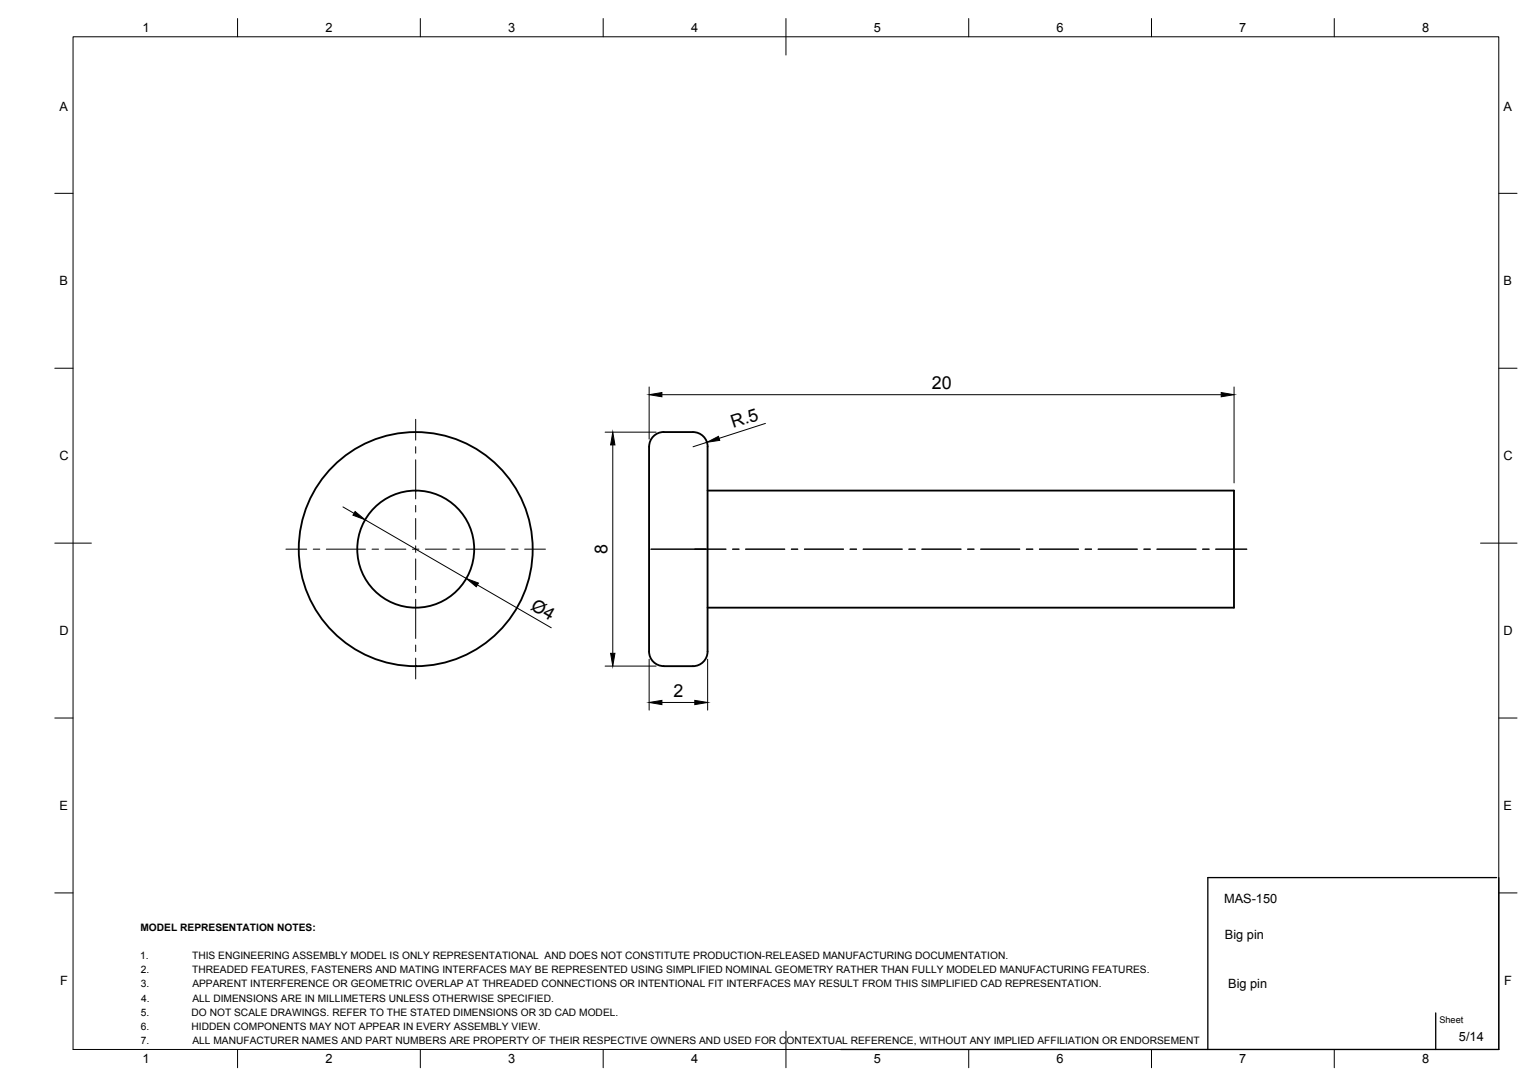
ISO-10303-21;
HEADER;
/* Generated by software containing ST-Developer
 * from STEP Tools, Inc. (www.steptools.com) 
 */

FILE_DESCRIPTION(
/* description */ ('STEP AP203'),
/* implementation_level */ '2;1');

FILE_NAME(
/* name */ 'Big pin.step',
/* time_stamp */ '2026-11-08T21:40:52-08:00',
/* author */ (''),
/* organization */ (''),
/* preprocessor_version */ 'ST-DEVELOPER v20.2',
/* originating_system */ 'Autodesk Translation Framework v15.17.0.0',
/* authorisation */ '');

FILE_SCHEMA (('AUTOMOTIVE_DESIGN { 1 0 10303 214 3 1 1 }'));
ENDSEC;

DATA;
#10=MECHANICAL_DESIGN_GEOMETRIC_PRESENTATION_REPRESENTATION('',(#192),#12137);
#170=SHAPE_REPRESENTATION_RELATIONSHIP('SRR','None',#12194,#181);
#181=ADVANCED_BREP_SHAPE_REPRESENTATION('',(#203),#12135);
#192=STYLED_ITEM('',(#12253),#203);
#203=MANIFOLD_SOLID_BREP('Body1',#1837);
#227=FACE_BOUND('',#723,.T.);
#269=PLANE('',#2128);
#270=PLANE('',#2129);
#271=PLANE('',#2130);
#358=LINE('',#12052,#452);
#359=LINE('',#12055,#453);
#452=VECTOR('',#2572,2.);
#453=VECTOR('',#2577,4.);
#484=CYLINDRICAL_SURFACE('',#2124,2.);
#485=CYLINDRICAL_SURFACE('',#2127,4.);
#585=FACE_OUTER_BOUND('',#717,.T.);
#586=FACE_OUTER_BOUND('',#718,.T.);
#587=FACE_OUTER_BOUND('',#719,.T.);
#588=FACE_OUTER_BOUND('',#720,.T.);
#589=FACE_OUTER_BOUND('',#721,.T.);
#590=FACE_OUTER_BOUND('',#722,.T.);
#591=FACE_OUTER_BOUND('',#724,.T.);
#717=EDGE_LOOP('',(#1651,#1652,#1653,#1654));
#718=EDGE_LOOP('',(#1655,#1656,#1657,#1658));
#719=EDGE_LOOP('',(#1659,#1660,#1661,#1662));
#720=EDGE_LOOP('',(#1663,#1664,#1665,#1666));
#721=EDGE_LOOP('',(#1667));
#722=EDGE_LOOP('',(#1668));
#723=EDGE_LOOP('',(#1669));
#724=EDGE_LOOP('',(#1670));
#808=CIRCLE('',#2117,3.5);
#809=CIRCLE('',#2118,0.5);
#810=CIRCLE('',#2119,4.);
#811=CIRCLE('',#2121,4.);
#812=CIRCLE('',#2122,0.5);
#813=CIRCLE('',#2123,3.5);
#814=CIRCLE('',#2125,2.);
#815=CIRCLE('',#2126,2.);
#963=VERTEX_POINT('',#12037);
#964=VERTEX_POINT('',#12039);
#965=VERTEX_POINT('',#12043);
#966=VERTEX_POINT('',#12045);
#967=VERTEX_POINT('',#12049);
#968=VERTEX_POINT('',#12051);
#1195=EDGE_CURVE('',#963,#963,#808,.T.);
#1196=EDGE_CURVE('',#963,#964,#809,.T.);
#1197=EDGE_CURVE('',#964,#964,#810,.T.);
#1198=EDGE_CURVE('',#965,#965,#811,.T.);
#1199=EDGE_CURVE('',#965,#966,#812,.T.);
#1200=EDGE_CURVE('',#966,#966,#813,.T.);
#1201=EDGE_CURVE('',#967,#967,#814,.T.);
#1202=EDGE_CURVE('',#967,#968,#358,.T.);
#1203=EDGE_CURVE('',#968,#968,#815,.T.);
#1204=EDGE_CURVE('',#964,#965,#359,.T.);
#1651=ORIENTED_EDGE('',*,*,#1195,.F.);
#1652=ORIENTED_EDGE('',*,*,#1196,.T.);
#1653=ORIENTED_EDGE('',*,*,#1197,.F.);
#1654=ORIENTED_EDGE('',*,*,#1196,.F.);
#1655=ORIENTED_EDGE('',*,*,#1198,.F.);
#1656=ORIENTED_EDGE('',*,*,#1199,.T.);
#1657=ORIENTED_EDGE('',*,*,#1200,.F.);
#1658=ORIENTED_EDGE('',*,*,#1199,.F.);
#1659=ORIENTED_EDGE('',*,*,#1201,.T.);
#1660=ORIENTED_EDGE('',*,*,#1202,.T.);
#1661=ORIENTED_EDGE('',*,*,#1203,.F.);
#1662=ORIENTED_EDGE('',*,*,#1202,.F.);
#1663=ORIENTED_EDGE('',*,*,#1197,.T.);
#1664=ORIENTED_EDGE('',*,*,#1204,.T.);
#1665=ORIENTED_EDGE('',*,*,#1198,.T.);
#1666=ORIENTED_EDGE('',*,*,#1204,.F.);
#1667=ORIENTED_EDGE('',*,*,#1200,.T.);
#1668=ORIENTED_EDGE('',*,*,#1195,.T.);
#1669=ORIENTED_EDGE('',*,*,#1201,.F.);
#1670=ORIENTED_EDGE('',*,*,#1203,.T.);
#1716=TOROIDAL_SURFACE('',#2116,3.5,0.5);
#1717=TOROIDAL_SURFACE('',#2120,3.5,0.5);
#1813=ADVANCED_FACE('',(#585),#1716,.T.);
#1814=ADVANCED_FACE('',(#586),#1717,.T.);
#1815=ADVANCED_FACE('',(#587),#484,.T.);
#1816=ADVANCED_FACE('',(#588),#485,.T.);
#1817=ADVANCED_FACE('',(#589),#269,.F.);
#1818=ADVANCED_FACE('',(#590,#227),#270,.T.);
#1819=ADVANCED_FACE('',(#591),#271,.T.);
#1837=CLOSED_SHELL('',(#1813,#1814,#1815,#1816,#1817,#1818,#1819));
#2115=AXIS2_PLACEMENT_3D('',#12035,#2550,#2551);
#2116=AXIS2_PLACEMENT_3D('',#12036,#2552,#2553);
#2117=AXIS2_PLACEMENT_3D('',#12038,#2554,#2555);
#2118=AXIS2_PLACEMENT_3D('',#12040,#2556,#2557);
#2119=AXIS2_PLACEMENT_3D('',#12041,#2558,#2559);
#2120=AXIS2_PLACEMENT_3D('',#12042,#2560,#2561);
#2121=AXIS2_PLACEMENT_3D('',#12044,#2562,#2563);
#2122=AXIS2_PLACEMENT_3D('',#12046,#2564,#2565);
#2123=AXIS2_PLACEMENT_3D('',#12047,#2566,#2567);
#2124=AXIS2_PLACEMENT_3D('',#12048,#2568,#2569);
#2125=AXIS2_PLACEMENT_3D('',#12050,#2570,#2571);
#2126=AXIS2_PLACEMENT_3D('',#12053,#2573,#2574);
#2127=AXIS2_PLACEMENT_3D('',#12054,#2575,#2576);
#2128=AXIS2_PLACEMENT_3D('',#12056,#2578,#2579);
#2129=AXIS2_PLACEMENT_3D('',#12057,#2580,#2581);
#2130=AXIS2_PLACEMENT_3D('',#12058,#2582,#2583);
#2550=DIRECTION('axis',(0.,0.,1.));
#2551=DIRECTION('refdir',(1.,0.,0.));
#2552=DIRECTION('center_axis',(-4.27556447653966E-32,1.97215226305253E-31,
1.));
#2553=DIRECTION('ref_axis',(1.,1.68641283164694E-62,0.));
#2554=DIRECTION('center_axis',(-4.27556447653966E-32,1.97215226305253E-31,
1.));
#2555=DIRECTION('ref_axis',(1.,1.76237737361302E-62,4.27556447653966E-32));
#2556=DIRECTION('center_axis',(1.22464679914735E-16,-1.,1.97215226305253E-31));
#2557=DIRECTION('ref_axis',(-1.,-1.22464679914735E-16,0.));
#2558=DIRECTION('center_axis',(4.27556447653966E-32,-1.97215226305253E-31,
-1.));
#2559=DIRECTION('ref_axis',(1.,8.88178419700125E-16,4.27556447653964E-32));
#2560=DIRECTION('center_axis',(-4.27556447653966E-32,1.97215226305253E-31,
1.));
#2561=DIRECTION('ref_axis',(1.,1.68641283164694E-62,0.));
#2562=DIRECTION('center_axis',(-4.27556447653966E-32,1.97215226305253E-31,
1.));
#2563=DIRECTION('ref_axis',(1.,8.4320641582347E-63,4.27556447653966E-32));
#2564=DIRECTION('center_axis',(1.22464679914735E-16,-1.,1.97215226305253E-31));
#2565=DIRECTION('ref_axis',(-1.,-1.22464679914735E-16,0.));
#2566=DIRECTION('center_axis',(4.27556447653966E-32,-1.97215226305253E-31,
-1.));
#2567=DIRECTION('ref_axis',(1.,8.4320641582347E-63,4.27556447653966E-32));
#2568=DIRECTION('center_axis',(4.27556447653966E-32,-1.97215226305253E-31,
-1.));
#2569=DIRECTION('ref_axis',(-1.,-8.4320641582347E-63,-4.27556447653966E-32));
#2570=DIRECTION('center_axis',(-4.27556447653966E-32,1.97215226305253E-31,
1.));
#2571=DIRECTION('ref_axis',(1.,1.76237737361302E-62,4.27556447653966E-32));
#2572=DIRECTION('',(-4.27556447653966E-32,1.97215226305253E-31,1.));
#2573=DIRECTION('center_axis',(-4.27556447653966E-32,1.97215226305253E-31,
1.));
#2574=DIRECTION('ref_axis',(1.,8.4320641582347E-63,4.27556447653966E-32));
#2575=DIRECTION('center_axis',(-4.27556447653966E-32,1.97215226305253E-31,
1.));
#2576=DIRECTION('ref_axis',(1.,8.4320641582347E-63,4.27556447653966E-32));
#2577=DIRECTION('',(4.27556447653966E-32,-1.97215226305253E-31,-1.));
#2578=DIRECTION('center_axis',(4.66075046541711E-32,1.97215226305253E-31,
1.));
#2579=DIRECTION('ref_axis',(1.,1.18072616964182E-79,-4.66075046541711E-32));
#2580=DIRECTION('center_axis',(4.66075046541711E-32,1.97215226305253E-31,
1.));
#2581=DIRECTION('ref_axis',(1.,1.18072616964182E-79,-4.66075046541711E-32));
#2582=DIRECTION('center_axis',(4.66075046541711E-32,1.97215226305253E-31,
1.));
#2583=DIRECTION('ref_axis',(1.,1.18072616964182E-79,-4.66075046541711E-32));
#12035=CARTESIAN_POINT('',(0.,0.,0.));
#12036=CARTESIAN_POINT('Origin',(0.,0.,-0.5));
#12037=CARTESIAN_POINT('',(-3.5,-4.28626379701574E-16,-7.48223783394441E-32));
#12038=CARTESIAN_POINT('Origin',(0.,0.,0.));
#12039=CARTESIAN_POINT('',(-4.,-4.89858719658941E-16,-0.5));
#12040=CARTESIAN_POINT('Origin',(-3.5,-4.28626379701574E-16,-0.5));
#12041=CARTESIAN_POINT('Origin',(0.,0.,-0.5));
#12042=CARTESIAN_POINT('Origin',(0.,0.,-1.5));
#12043=CARTESIAN_POINT('',(-4.,-4.89858719658941E-16,-1.5));
#12044=CARTESIAN_POINT('Origin',(0.,0.,-1.5));
#12045=CARTESIAN_POINT('',(-3.5,-4.28626379701574E-16,-2.));
#12046=CARTESIAN_POINT('Origin',(-3.5,-4.28626379701574E-16,-1.5));
#12047=CARTESIAN_POINT('Origin',(0.,-6.93889390390723E-15,-2.));
#12048=CARTESIAN_POINT('Origin',(0.,0.,18.));
#12049=CARTESIAN_POINT('',(2.,-2.44929359829474E-16,0.));
#12050=CARTESIAN_POINT('Origin',(0.,0.,0.));
#12051=CARTESIAN_POINT('',(2.,-2.44929359829471E-16,18.));
#12052=CARTESIAN_POINT('',(2.,-2.44929359829471E-16,18.));
#12053=CARTESIAN_POINT('Origin',(0.,0.,18.));
#12054=CARTESIAN_POINT('Origin',(0.,-6.93889390390723E-15,-2.));
#12055=CARTESIAN_POINT('',(-4.,-7.42875262356617E-15,-2.));
#12056=CARTESIAN_POINT('Origin',(0.,-6.93889390390723E-15,-2.));
#12057=CARTESIAN_POINT('Origin',(0.,0.,0.));
#12058=CARTESIAN_POINT('Origin',(0.,0.,18.));
#12121=UNCERTAINTY_MEASURE_WITH_UNIT(LENGTH_MEASURE(0.01),#12138,
'DISTANCE_ACCURACY_VALUE',
'Maximum model space distance between geometric entities at asserted c
onnectivities');
#12123=UNCERTAINTY_MEASURE_WITH_UNIT(LENGTH_MEASURE(0.01),#12138,
'DISTANCE_ACCURACY_VALUE',
'Maximum model space distance between geometric entities at asserted c
onnectivities');
#12135=(
GEOMETRIC_REPRESENTATION_CONTEXT(3)
GLOBAL_UNCERTAINTY_ASSIGNED_CONTEXT((#12121))
GLOBAL_UNIT_ASSIGNED_CONTEXT((#12138,#12140,#12141))
REPRESENTATION_CONTEXT('','3D')
);
#12137=(
GEOMETRIC_REPRESENTATION_CONTEXT(3)
GLOBAL_UNCERTAINTY_ASSIGNED_CONTEXT((#12123))
GLOBAL_UNIT_ASSIGNED_CONTEXT((#12138,#12140,#12141))
REPRESENTATION_CONTEXT('','3D')
);
#12138=(
LENGTH_UNIT()
NAMED_UNIT(*)
SI_UNIT(.MILLI.,.METRE.)
);
#12140=(
NAMED_UNIT(*)
PLANE_ANGLE_UNIT()
SI_UNIT($,.RADIAN.)
);
#12141=(
NAMED_UNIT(*)
SI_UNIT($,.STERADIAN.)
SOLID_ANGLE_UNIT()
);
#12153=SHAPE_DEFINITION_REPRESENTATION(#12169,#12194);
#12169=PRODUCT_DEFINITION_SHAPE('',$,#12208);
#12194=SHAPE_REPRESENTATION('',(#2115),#12135);
#12196=PRODUCT_DEFINITION_CONTEXT('part definition',#12237,'design');
#12208=PRODUCT_DEFINITION('Big pin','Big pin',#12221,#12196);
#12221=PRODUCT_DEFINITION_FORMATION('',$,#12250);
#12237=APPLICATION_CONTEXT(
'Core Data for Automotive Mechanical Design Process');
#12238=PRODUCT_CONTEXT('part definition',#12237,'mechanical');
#12250=PRODUCT('Big pin','Big pin',$,(#12238));
#12253=PRESENTATION_STYLE_ASSIGNMENT((#12255));
#12255=SURFACE_STYLE_USAGE(.BOTH.,#12257);
#12257=SURFACE_SIDE_STYLE('',(#12259));
#12259=SURFACE_STYLE_FILL_AREA(#12261);
#12261=FILL_AREA_STYLE('Opaque(23,69,131)',(#12263));
#12263=FILL_AREA_STYLE_COLOUR('Opaque(23,69,131)',#12265);
#12265=COLOUR_RGB('Opaque(23,69,131)',0.0901960784313725,0.270588235294118,
0.513725490196078);
ENDSEC;
END-ISO-10303-21;
